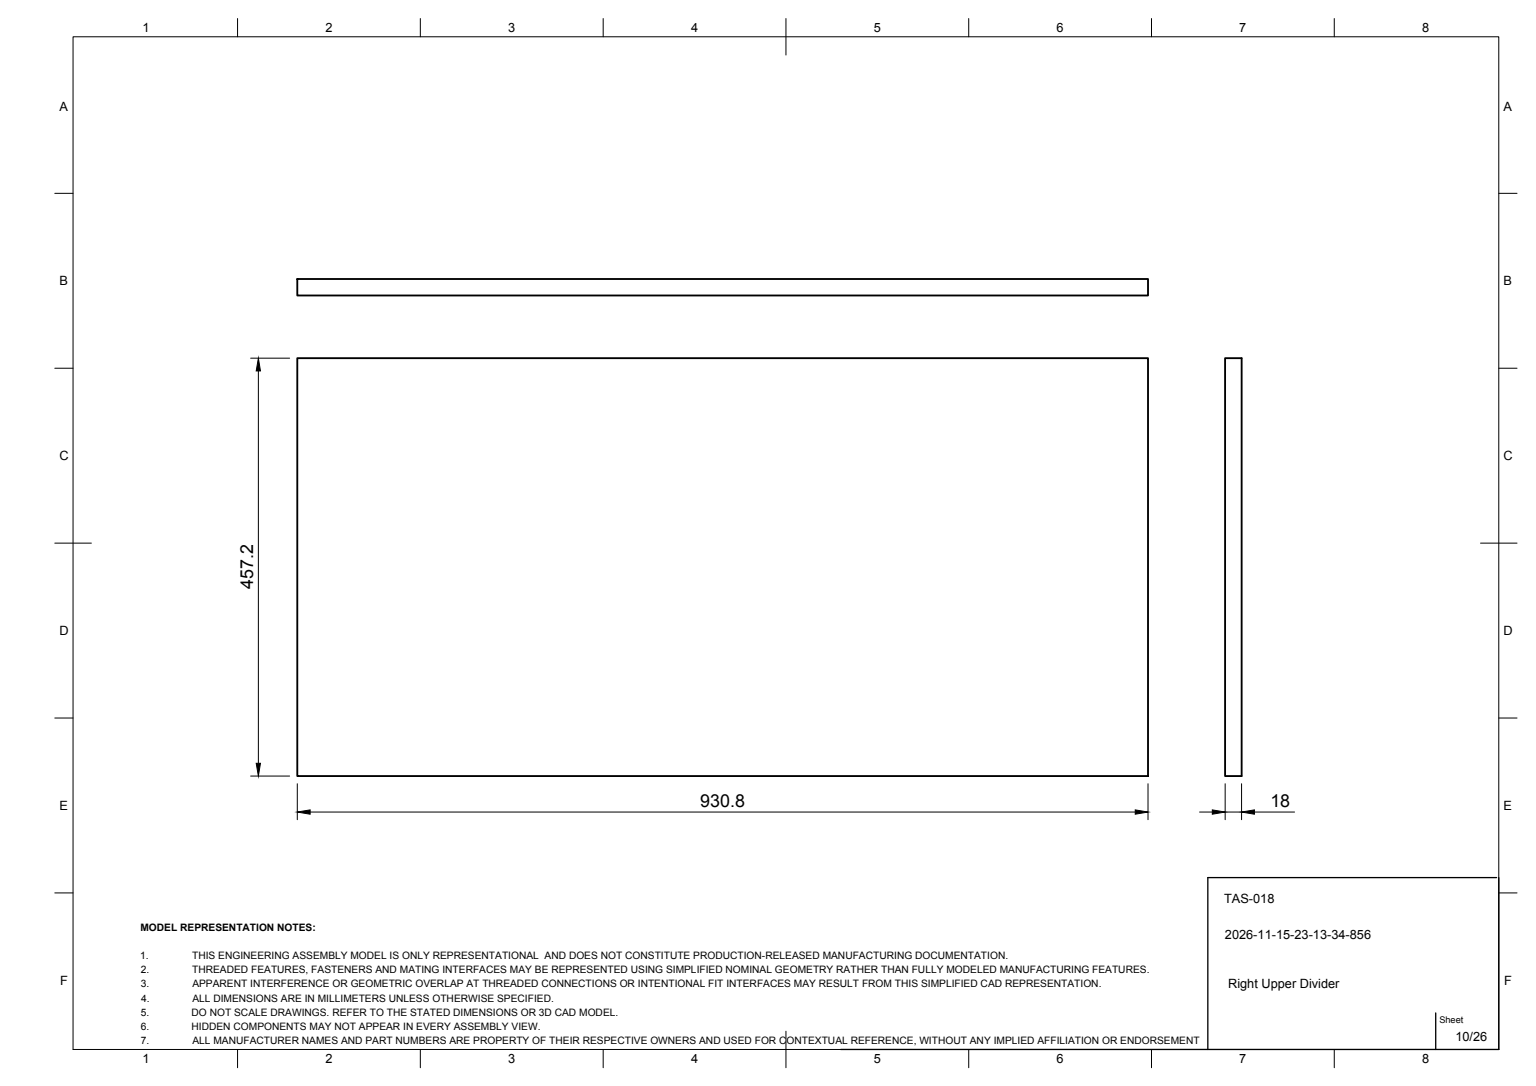
ISO-10303-21;
HEADER;
/* Generated by software containing ST-Developer
 * from STEP Tools, Inc. (www.steptools.com) 
 */

FILE_DESCRIPTION(
/* description */ (''),
/* implementation_level */ '2;1');

FILE_NAME(
/* name */ 'Right Upper Divider.step',
/* time_stamp */ '2026-11-15T15:17:57-08:00',
/* author */ (''),
/* organization */ (''),
/* preprocessor_version */ 'ST-DEVELOPER v20.2',
/* originating_system */ 'Autodesk Translation Framework v15.17.0.0',
/* authorisation */ '');

FILE_SCHEMA (('AUTOMOTIVE_DESIGN { 1 0 10303 214 3 1 1 }'));
ENDSEC;

DATA;
#10=MECHANICAL_DESIGN_GEOMETRIC_PRESENTATION_REPRESENTATION('',(#185),#3723);
#137=SHAPE_REPRESENTATION_RELATIONSHIP('SRR','None',#3818,#161);
#161=ADVANCED_BREP_SHAPE_REPRESENTATION('',(#209),#3707);
#185=STYLED_ITEM('',(#3946),#209);
#209=MANIFOLD_SOLID_BREP('Body1',#2033);
#270=FACE_OUTER_BOUND('',#396,.T.);
#271=FACE_OUTER_BOUND('',#397,.T.);
#272=FACE_OUTER_BOUND('',#398,.T.);
#273=FACE_OUTER_BOUND('',#399,.T.);
#274=FACE_OUTER_BOUND('',#400,.T.);
#275=FACE_OUTER_BOUND('',#401,.T.);
#396=EDGE_LOOP('',(#1485,#1486,#1487,#1488));
#397=EDGE_LOOP('',(#1489,#1490,#1491,#1492));
#398=EDGE_LOOP('',(#1493,#1494,#1495,#1496));
#399=EDGE_LOOP('',(#1497,#1498,#1499,#1500));
#400=EDGE_LOOP('',(#1501,#1502,#1503,#1504));
#401=EDGE_LOOP('',(#1505,#1506,#1507,#1508));
#562=LINE('',#3308,#784);
#563=LINE('',#3310,#785);
#564=LINE('',#3312,#786);
#565=LINE('',#3313,#787);
#566=LINE('',#3316,#788);
#567=LINE('',#3318,#789);
#568=LINE('',#3319,#790);
#569=LINE('',#3322,#791);
#570=LINE('',#3324,#792);
#571=LINE('',#3325,#793);
#572=LINE('',#3327,#794);
#573=LINE('',#3328,#795);
#784=VECTOR('',#2708,36.6456692913386);
#785=VECTOR('',#2709,18.);
#786=VECTOR('',#2710,36.6456692913386);
#787=VECTOR('',#2711,18.);
#788=VECTOR('',#2714,0.708661417322839);
#789=VECTOR('',#2715,0.708661417322839);
#790=VECTOR('',#2716,18.);
#791=VECTOR('',#2719,36.6456692913386);
#792=VECTOR('',#2720,36.6456692913386);
#793=VECTOR('',#2721,18.);
#794=VECTOR('',#2724,0.708661417322839);
#795=VECTOR('',#2725,0.708661417322839);
#979=VERTEX_POINT('',#3306);
#980=VERTEX_POINT('',#3307);
#981=VERTEX_POINT('',#3309);
#982=VERTEX_POINT('',#3311);
#983=VERTEX_POINT('',#3315);
#984=VERTEX_POINT('',#3317);
#985=VERTEX_POINT('',#3321);
#986=VERTEX_POINT('',#3323);
#1164=EDGE_CURVE('',#979,#980,#562,.T.);
#1165=EDGE_CURVE('',#979,#981,#563,.T.);
#1166=EDGE_CURVE('',#981,#982,#564,.T.);
#1167=EDGE_CURVE('',#980,#982,#565,.T.);
#1168=EDGE_CURVE('',#980,#983,#566,.T.);
#1169=EDGE_CURVE('',#982,#984,#567,.T.);
#1170=EDGE_CURVE('',#983,#984,#568,.T.);
#1171=EDGE_CURVE('',#983,#985,#569,.T.);
#1172=EDGE_CURVE('',#984,#986,#570,.T.);
#1173=EDGE_CURVE('',#985,#986,#571,.T.);
#1174=EDGE_CURVE('',#985,#979,#572,.T.);
#1175=EDGE_CURVE('',#986,#981,#573,.T.);
#1485=ORIENTED_EDGE('',*,*,#1164,.F.);
#1486=ORIENTED_EDGE('',*,*,#1165,.T.);
#1487=ORIENTED_EDGE('',*,*,#1166,.T.);
#1488=ORIENTED_EDGE('',*,*,#1167,.F.);
#1489=ORIENTED_EDGE('',*,*,#1168,.F.);
#1490=ORIENTED_EDGE('',*,*,#1167,.T.);
#1491=ORIENTED_EDGE('',*,*,#1169,.T.);
#1492=ORIENTED_EDGE('',*,*,#1170,.F.);
#1493=ORIENTED_EDGE('',*,*,#1171,.F.);
#1494=ORIENTED_EDGE('',*,*,#1170,.T.);
#1495=ORIENTED_EDGE('',*,*,#1172,.T.);
#1496=ORIENTED_EDGE('',*,*,#1173,.F.);
#1497=ORIENTED_EDGE('',*,*,#1174,.F.);
#1498=ORIENTED_EDGE('',*,*,#1173,.T.);
#1499=ORIENTED_EDGE('',*,*,#1175,.T.);
#1500=ORIENTED_EDGE('',*,*,#1165,.F.);
#1501=ORIENTED_EDGE('',*,*,#1166,.F.);
#1502=ORIENTED_EDGE('',*,*,#1175,.F.);
#1503=ORIENTED_EDGE('',*,*,#1172,.F.);
#1504=ORIENTED_EDGE('',*,*,#1169,.F.);
#1505=ORIENTED_EDGE('',*,*,#1174,.T.);
#1506=ORIENTED_EDGE('',*,*,#1164,.T.);
#1507=ORIENTED_EDGE('',*,*,#1168,.T.);
#1508=ORIENTED_EDGE('',*,*,#1171,.T.);
#1823=PLANE('',#2373);
#1824=PLANE('',#2374);
#1825=PLANE('',#2375);
#1826=PLANE('',#2376);
#1827=PLANE('',#2377);
#1828=PLANE('',#2378);
#1944=ADVANCED_FACE('',(#270),#1823,.F.);
#1945=ADVANCED_FACE('',(#271),#1824,.F.);
#1946=ADVANCED_FACE('',(#272),#1825,.F.);
#1947=ADVANCED_FACE('',(#273),#1826,.F.);
#1948=ADVANCED_FACE('',(#274),#1827,.F.);
#1949=ADVANCED_FACE('',(#275),#1828,.T.);
#2033=CLOSED_SHELL('',(#1944,#1945,#1946,#1947,#1948,#1949));
#2372=AXIS2_PLACEMENT_3D('',#3304,#2704,#2705);
#2373=AXIS2_PLACEMENT_3D('',#3305,#2706,#2707);
#2374=AXIS2_PLACEMENT_3D('',#3314,#2712,#2713);
#2375=AXIS2_PLACEMENT_3D('',#3320,#2717,#2718);
#2376=AXIS2_PLACEMENT_3D('',#3326,#2722,#2723);
#2377=AXIS2_PLACEMENT_3D('',#3329,#2726,#2727);
#2378=AXIS2_PLACEMENT_3D('',#3330,#2728,#2729);
#2704=DIRECTION('axis',(0.,0.,1.));
#2705=DIRECTION('refdir',(1.,0.,0.));
#2706=DIRECTION('center_axis',(1.,1.19276216655045E-16,0.));
#2707=DIRECTION('ref_axis',(0.,0.,-1.));
#2708=DIRECTION('',(1.52673557318457E-16,-1.,0.));
#2709=DIRECTION('',(0.,0.,-1.));
#2710=DIRECTION('',(1.52673557318457E-16,-1.,0.));
#2711=DIRECTION('',(0.,0.,-1.));
#2712=DIRECTION('center_axis',(0.,1.,0.));
#2713=DIRECTION('ref_axis',(0.,0.,1.));
#2714=DIRECTION('',(1.,0.,0.));
#2715=DIRECTION('',(1.,0.,0.));
#2716=DIRECTION('',(0.,0.,-1.));
#2717=DIRECTION('center_axis',(-1.,-1.19276216655045E-16,0.));
#2718=DIRECTION('ref_axis',(0.,0.,1.));
#2719=DIRECTION('',(-1.52673557318457E-16,1.,0.));
#2720=DIRECTION('',(-1.52673557318457E-16,1.,0.));
#2721=DIRECTION('',(0.,0.,-1.));
#2722=DIRECTION('center_axis',(0.,-1.,0.));
#2723=DIRECTION('ref_axis',(0.,0.,-1.));
#2724=DIRECTION('',(-1.,0.,0.));
#2725=DIRECTION('',(-1.,0.,0.));
#2726=DIRECTION('center_axis',(0.,0.,1.));
#2727=DIRECTION('ref_axis',(1.,0.,0.));
#2728=DIRECTION('center_axis',(0.,0.,1.));
#2729=DIRECTION('ref_axis',(1.,0.,0.));
#3304=CARTESIAN_POINT('',(0.,0.,0.));
#3305=CARTESIAN_POINT('Origin',(22.9370078740157,66.6456692913386,60.3603597227694));
#3306=CARTESIAN_POINT('',(22.9370078740157,66.6456692913386,18.7086614173228));
#3307=CARTESIAN_POINT('',(22.9370078740157,30.,18.7086614173228));
#3308=CARTESIAN_POINT('',(22.9370078740157,66.6456692913386,18.7086614173228));
#3309=CARTESIAN_POINT('',(22.9370078740157,66.6456692913386,0.708661417322834));
#3310=CARTESIAN_POINT('',(22.9370078740157,66.6456692913386,18.7086614173228));
#3311=CARTESIAN_POINT('',(22.9370078740157,30.,0.708661417322834));
#3312=CARTESIAN_POINT('',(22.9370078740157,66.6456692913386,0.708661417322834));
#3313=CARTESIAN_POINT('',(22.9370078740157,30.,18.7086614173228));
#3314=CARTESIAN_POINT('Origin',(22.9370078740157,30.,60.3603597227694));
#3315=CARTESIAN_POINT('',(23.6456692913386,30.,18.7086614173228));
#3316=CARTESIAN_POINT('',(22.9370078740157,30.,18.7086614173228));
#3317=CARTESIAN_POINT('',(23.6456692913386,30.,0.708661417322834));
#3318=CARTESIAN_POINT('',(22.9370078740157,30.,0.708661417322834));
#3319=CARTESIAN_POINT('',(23.6456692913386,30.,18.7086614173228));
#3320=CARTESIAN_POINT('Origin',(23.6456692913386,66.6456692913386,60.3603597227694));
#3321=CARTESIAN_POINT('',(23.6456692913386,66.6456692913386,18.7086614173228));
#3322=CARTESIAN_POINT('',(23.6456692913386,30.,18.7086614173228));
#3323=CARTESIAN_POINT('',(23.6456692913386,66.6456692913386,0.708661417322834));
#3324=CARTESIAN_POINT('',(23.6456692913386,30.,0.708661417322834));
#3325=CARTESIAN_POINT('',(23.6456692913386,66.6456692913386,18.7086614173228));
#3326=CARTESIAN_POINT('Origin',(22.9370078740157,66.6456692913386,60.3603597227694));
#3327=CARTESIAN_POINT('',(23.6456692913386,66.6456692913386,18.7086614173228));
#3328=CARTESIAN_POINT('',(23.6456692913386,66.6456692913386,0.708661417322834));
#3329=CARTESIAN_POINT('Origin',(0.,0.,0.708661417322834));
#3330=CARTESIAN_POINT('Origin',(0.,0.,18.7086614173228));
#3680=UNCERTAINTY_MEASURE_WITH_UNIT(LENGTH_MEASURE(0.000393700787401575),
#3725,'DISTANCE_ACCURACY_VALUE',
'Maximum model space distance between geometric entities at asserted c
onnectivities');
#3696=UNCERTAINTY_MEASURE_WITH_UNIT(LENGTH_MEASURE(0.000393700787401575),
#3725,'DISTANCE_ACCURACY_VALUE',
'Maximum model space distance between geometric entities at asserted c
onnectivities');
#3707=(
GEOMETRIC_REPRESENTATION_CONTEXT(3)
GLOBAL_UNCERTAINTY_ASSIGNED_CONTEXT((#3680))
GLOBAL_UNIT_ASSIGNED_CONTEXT((#3725,#3729,#3730))
REPRESENTATION_CONTEXT('','3D')
);
#3723=(
GEOMETRIC_REPRESENTATION_CONTEXT(3)
GLOBAL_UNCERTAINTY_ASSIGNED_CONTEXT((#3696))
GLOBAL_UNIT_ASSIGNED_CONTEXT((#3725,#3729,#3730))
REPRESENTATION_CONTEXT('','3D')
);
#3724=DIMENSIONAL_EXPONENTS(1.,0.,0.,0.,0.,0.,0.);
#3725=(
CONVERSION_BASED_UNIT('inch',#3728)
LENGTH_UNIT()
NAMED_UNIT(#3724)
);
#3726=(
LENGTH_UNIT()
NAMED_UNIT(*)
SI_UNIT(.MILLI.,.METRE.)
);
#3728=LENGTH_MEASURE_WITH_UNIT(LENGTH_MEASURE(25.4),#3726);
#3729=(
NAMED_UNIT(*)
PLANE_ANGLE_UNIT()
SI_UNIT($,.RADIAN.)
);
#3730=(
NAMED_UNIT(*)
SI_UNIT($,.STERADIAN.)
SOLID_ANGLE_UNIT()
);
#3741=SHAPE_DEFINITION_REPRESENTATION(#3768,#3818);
#3768=PRODUCT_DEFINITION_SHAPE('',$,#3845);
#3818=SHAPE_REPRESENTATION('',(#2372),#3707);
#3834=PRODUCT_DEFINITION_CONTEXT('part definition',#3914,'design');
#3845=PRODUCT_DEFINITION('2026-11-15-23-13-34-856',
'Right Upper Divider',#3871,#3834);
#3871=PRODUCT_DEFINITION_FORMATION('',$,#3926);
#3914=APPLICATION_CONTEXT(
'Core Data for Automotive Mechanical Design Process');
#3915=PRODUCT_CONTEXT('part definition',#3914,'mechanical');
#3926=PRODUCT('2026-11-15-23-13-34-856','Right Upper Divider',$,(#3915));
#3946=PRESENTATION_STYLE_ASSIGNMENT((#3954));
#3954=SURFACE_STYLE_USAGE(.BOTH.,#3962);
#3962=SURFACE_SIDE_STYLE('',(#3970));
#3970=SURFACE_STYLE_FILL_AREA(#3978);
#3978=FILL_AREA_STYLE('Gray',(#3986));
#3986=FILL_AREA_STYLE_COLOUR('Gray',#3994);
#3994=COLOUR_RGB('Gray',0.501960784313725,0.501960784313725,0.501960784313725);
ENDSEC;
END-ISO-10303-21;
